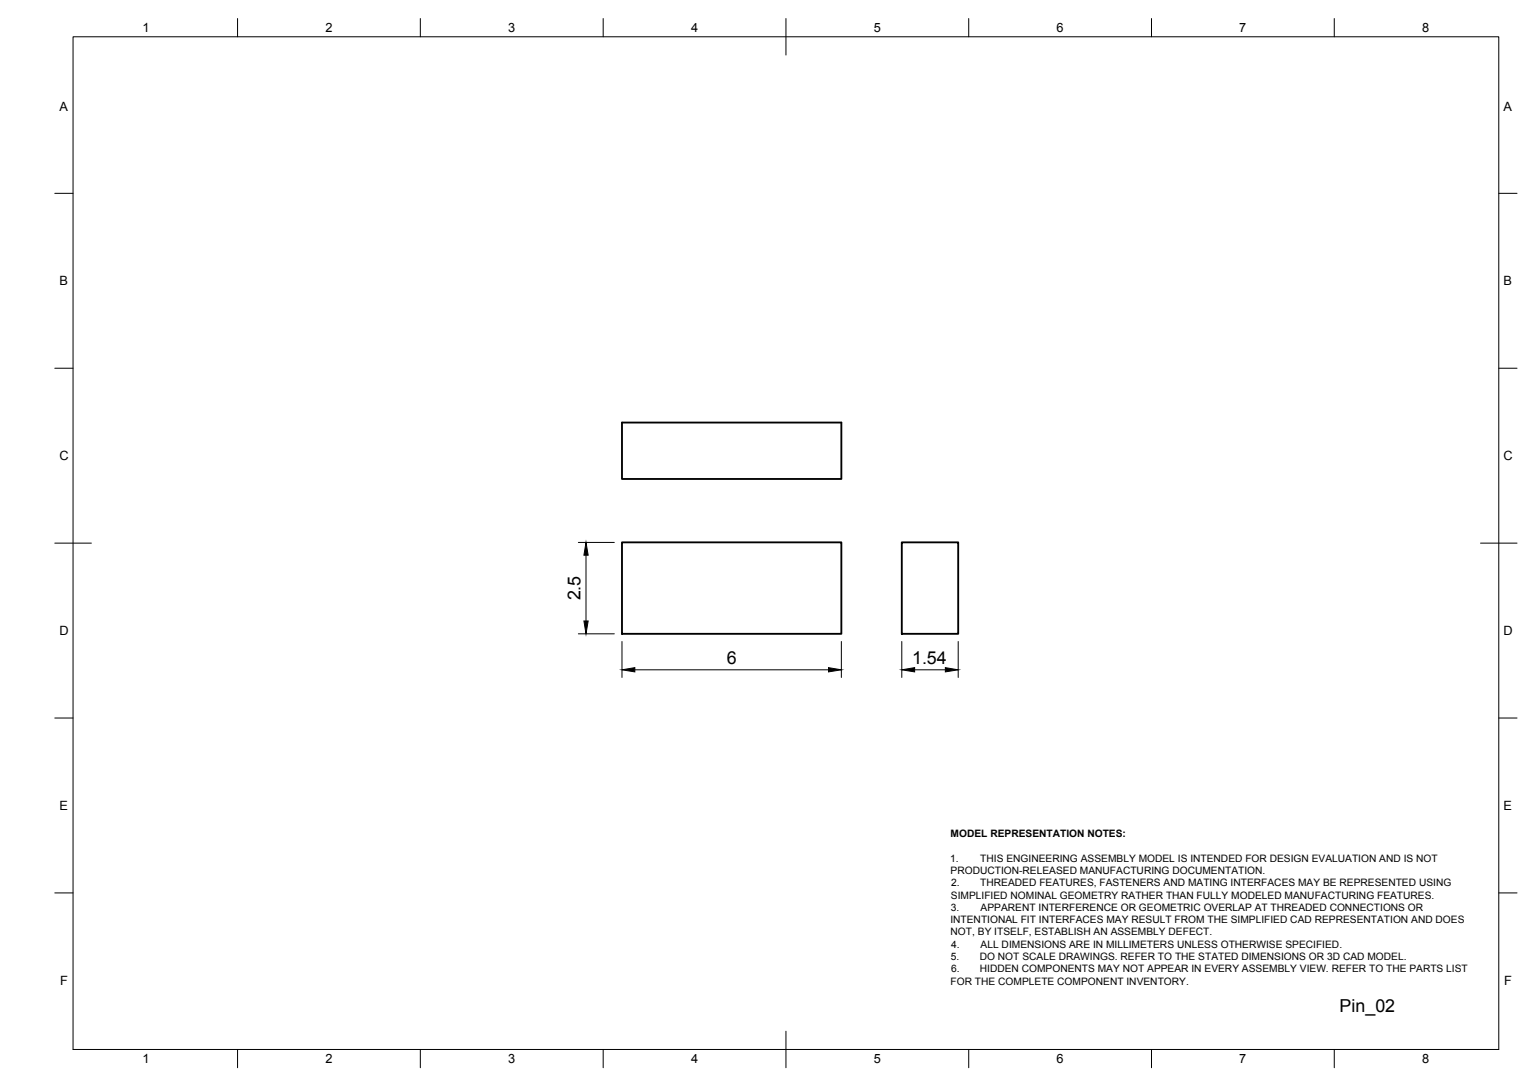
ISO-10303-21;
HEADER;
/* Generated by software containing ST-Developer
 * from STEP Tools, Inc. (www.steptools.com) 
 */

FILE_DESCRIPTION(
/* description */ (''),
/* implementation_level */ '2;1');

FILE_NAME(
/* name */ 'Pin_02.step',
/* time_stamp */ '2026-10-05T22:24:12-07:00',
/* author */ (''),
/* organization */ (''),
/* preprocessor_version */ 'ST-DEVELOPER v20.2',
/* originating_system */ 'Autodesk Translation Framework v15.15.0.0',
/* authorisation */ '');

FILE_SCHEMA (('AUTOMOTIVE_DESIGN { 1 0 10303 214 3 1 1 }'));
ENDSEC;

DATA;
#10=MECHANICAL_DESIGN_GEOMETRIC_PRESENTATION_REPRESENTATION('',(#57),#2116);
#43=SHAPE_REPRESENTATION_RELATIONSHIP('SRR','None',#2149,#50);
#50=ADVANCED_BREP_SHAPE_REPRESENTATION('',(#64),#2113);
#57=STYLED_ITEM('',(#2192),#64);
#64=MANIFOLD_SOLID_BREP('Body1',#1151);
#113=PLANE('',#1322);
#114=PLANE('',#1323);
#115=PLANE('',#1324);
#116=PLANE('',#1325);
#117=PLANE('',#1326);
#118=PLANE('',#1327);
#179=FACE_OUTER_BOUND('',#254,.T.);
#180=FACE_OUTER_BOUND('',#255,.T.);
#181=FACE_OUTER_BOUND('',#256,.T.);
#182=FACE_OUTER_BOUND('',#257,.T.);
#183=FACE_OUTER_BOUND('',#258,.T.);
#184=FACE_OUTER_BOUND('',#259,.T.);
#254=EDGE_LOOP('',(#991,#992,#993,#994));
#255=EDGE_LOOP('',(#995,#996,#997,#998));
#256=EDGE_LOOP('',(#999,#1000,#1001,#1002));
#257=EDGE_LOOP('',(#1003,#1004,#1005,#1006));
#258=EDGE_LOOP('',(#1007,#1008,#1009,#1010));
#259=EDGE_LOOP('',(#1011,#1012,#1013,#1014));
#346=LINE('',#2009,#451);
#347=LINE('',#2011,#452);
#348=LINE('',#2013,#453);
#349=LINE('',#2014,#454);
#350=LINE('',#2017,#455);
#351=LINE('',#2019,#456);
#352=LINE('',#2020,#457);
#353=LINE('',#2023,#458);
#354=LINE('',#2025,#459);
#355=LINE('',#2026,#460);
#356=LINE('',#2028,#461);
#357=LINE('',#2029,#462);
#451=VECTOR('',#1606,10.);
#452=VECTOR('',#1607,10.);
#453=VECTOR('',#1608,10.);
#454=VECTOR('',#1609,10.);
#455=VECTOR('',#1612,10.);
#456=VECTOR('',#1613,10.);
#457=VECTOR('',#1614,10.);
#458=VECTOR('',#1617,10.);
#459=VECTOR('',#1618,10.);
#460=VECTOR('',#1619,10.);
#461=VECTOR('',#1622,10.);
#462=VECTOR('',#1623,10.);
#599=VERTEX_POINT('',#2007);
#600=VERTEX_POINT('',#2008);
#601=VERTEX_POINT('',#2010);
#602=VERTEX_POINT('',#2012);
#603=VERTEX_POINT('',#2016);
#604=VERTEX_POINT('',#2018);
#605=VERTEX_POINT('',#2022);
#606=VERTEX_POINT('',#2024);
#734=EDGE_CURVE('',#599,#600,#346,.T.);
#735=EDGE_CURVE('',#600,#601,#347,.T.);
#736=EDGE_CURVE('',#601,#602,#348,.T.);
#737=EDGE_CURVE('',#599,#602,#349,.T.);
#738=EDGE_CURVE('',#600,#603,#350,.T.);
#739=EDGE_CURVE('',#603,#604,#351,.T.);
#740=EDGE_CURVE('',#604,#601,#352,.T.);
#741=EDGE_CURVE('',#605,#603,#353,.T.);
#742=EDGE_CURVE('',#605,#606,#354,.T.);
#743=EDGE_CURVE('',#606,#604,#355,.T.);
#744=EDGE_CURVE('',#599,#605,#356,.T.);
#745=EDGE_CURVE('',#602,#606,#357,.T.);
#991=ORIENTED_EDGE('',*,*,#734,.T.);
#992=ORIENTED_EDGE('',*,*,#735,.T.);
#993=ORIENTED_EDGE('',*,*,#736,.T.);
#994=ORIENTED_EDGE('',*,*,#737,.F.);
#995=ORIENTED_EDGE('',*,*,#738,.T.);
#996=ORIENTED_EDGE('',*,*,#739,.T.);
#997=ORIENTED_EDGE('',*,*,#740,.T.);
#998=ORIENTED_EDGE('',*,*,#735,.F.);
#999=ORIENTED_EDGE('',*,*,#741,.F.);
#1000=ORIENTED_EDGE('',*,*,#742,.T.);
#1001=ORIENTED_EDGE('',*,*,#743,.T.);
#1002=ORIENTED_EDGE('',*,*,#739,.F.);
#1003=ORIENTED_EDGE('',*,*,#744,.F.);
#1004=ORIENTED_EDGE('',*,*,#737,.T.);
#1005=ORIENTED_EDGE('',*,*,#745,.T.);
#1006=ORIENTED_EDGE('',*,*,#742,.F.);
#1007=ORIENTED_EDGE('',*,*,#745,.F.);
#1008=ORIENTED_EDGE('',*,*,#736,.F.);
#1009=ORIENTED_EDGE('',*,*,#740,.F.);
#1010=ORIENTED_EDGE('',*,*,#743,.F.);
#1011=ORIENTED_EDGE('',*,*,#744,.T.);
#1012=ORIENTED_EDGE('',*,*,#741,.T.);
#1013=ORIENTED_EDGE('',*,*,#738,.F.);
#1014=ORIENTED_EDGE('',*,*,#734,.F.);
#1128=ADVANCED_FACE('',(#179),#113,.F.);
#1129=ADVANCED_FACE('',(#180),#114,.F.);
#1130=ADVANCED_FACE('',(#181),#115,.F.);
#1131=ADVANCED_FACE('',(#182),#116,.F.);
#1132=ADVANCED_FACE('',(#183),#117,.F.);
#1133=ADVANCED_FACE('',(#184),#118,.T.);
#1151=CLOSED_SHELL('',(#1128,#1129,#1130,#1131,#1132,#1133));
#1321=AXIS2_PLACEMENT_3D('',#2005,#1602,#1603);
#1322=AXIS2_PLACEMENT_3D('',#2006,#1604,#1605);
#1323=AXIS2_PLACEMENT_3D('',#2015,#1610,#1611);
#1324=AXIS2_PLACEMENT_3D('',#2021,#1615,#1616);
#1325=AXIS2_PLACEMENT_3D('',#2027,#1620,#1621);
#1326=AXIS2_PLACEMENT_3D('',#2030,#1624,#1625);
#1327=AXIS2_PLACEMENT_3D('',#2031,#1626,#1627);
#1602=DIRECTION('axis',(0.,0.,1.));
#1603=DIRECTION('refdir',(1.,0.,0.));
#1604=DIRECTION('center_axis',(0.,0.,-1.));
#1605=DIRECTION('ref_axis',(-1.,0.,0.));
#1606=DIRECTION('',(1.,0.,0.));
#1607=DIRECTION('',(0.,1.,0.));
#1608=DIRECTION('',(-1.,0.,0.));
#1609=DIRECTION('',(0.,1.,0.));
#1610=DIRECTION('center_axis',(-1.,0.,0.));
#1611=DIRECTION('ref_axis',(0.,0.,1.));
#1612=DIRECTION('',(0.,0.,-1.));
#1613=DIRECTION('',(0.,1.,0.));
#1614=DIRECTION('',(0.,0.,1.));
#1615=DIRECTION('center_axis',(0.,0.,1.));
#1616=DIRECTION('ref_axis',(1.,0.,0.));
#1617=DIRECTION('',(1.,0.,0.));
#1618=DIRECTION('',(0.,1.,0.));
#1619=DIRECTION('',(1.,0.,0.));
#1620=DIRECTION('center_axis',(1.,0.,0.));
#1621=DIRECTION('ref_axis',(0.,0.,-1.));
#1622=DIRECTION('',(0.,0.,-1.));
#1623=DIRECTION('',(0.,0.,-1.));
#1624=DIRECTION('center_axis',(0.,-1.,0.));
#1625=DIRECTION('ref_axis',(0.,0.,-1.));
#1626=DIRECTION('center_axis',(0.,-1.,0.));
#1627=DIRECTION('ref_axis',(1.,0.,0.));
#2005=CARTESIAN_POINT('',(0.,0.,0.));
#2006=CARTESIAN_POINT('Origin',(3.25,10.,6.84122918275927));
#2007=CARTESIAN_POINT('',(0.75,10.,6.84122918275927));
#2008=CARTESIAN_POINT('',(3.25,10.,6.84122918275927));
#2009=CARTESIAN_POINT('',(0.75,10.,6.84122918275927));
#2010=CARTESIAN_POINT('',(3.25,16.,6.84122918275927));
#2011=CARTESIAN_POINT('',(3.25,10.,6.84122918275927));
#2012=CARTESIAN_POINT('',(0.75,16.,6.84122918275927));
#2013=CARTESIAN_POINT('',(0.75,16.,6.84122918275927));
#2014=CARTESIAN_POINT('',(0.75,10.,6.84122918275927));
#2015=CARTESIAN_POINT('Origin',(3.25,10.,5.29967103839267));
#2016=CARTESIAN_POINT('',(3.25,10.,5.29967103839267));
#2017=CARTESIAN_POINT('',(3.25,10.,8.32461990770089));
#2018=CARTESIAN_POINT('',(3.25,16.,5.29967103839267));
#2019=CARTESIAN_POINT('',(3.25,10.,5.29967103839267));
#2020=CARTESIAN_POINT('',(3.25,16.,8.32461990770089));
#2021=CARTESIAN_POINT('Origin',(0.75,10.,5.29967103839267));
#2022=CARTESIAN_POINT('',(0.75,10.,5.29967103839267));
#2023=CARTESIAN_POINT('',(0.75,10.,5.29967103839267));
#2024=CARTESIAN_POINT('',(0.75,16.,5.29967103839267));
#2025=CARTESIAN_POINT('',(0.75,10.,5.29967103839267));
#2026=CARTESIAN_POINT('',(0.75,16.,5.29967103839267));
#2027=CARTESIAN_POINT('Origin',(0.75,10.,6.84122918275927));
#2028=CARTESIAN_POINT('',(0.75,10.,5.79967103839267));
#2029=CARTESIAN_POINT('',(0.75,16.,5.79967103839267));
#2030=CARTESIAN_POINT('Origin',(2.,16.,6.07045011057597));
#2031=CARTESIAN_POINT('Origin',(2.,10.,6.07045011057597));
#2104=UNCERTAINTY_MEASURE_WITH_UNIT(LENGTH_MEASURE(0.01),#2117,
'DISTANCE_ACCURACY_VALUE',
'Maximum model space distance between geometric entities at asserted c
onnectivities');
#2107=UNCERTAINTY_MEASURE_WITH_UNIT(LENGTH_MEASURE(0.01),#2117,
'DISTANCE_ACCURACY_VALUE',
'Maximum model space distance between geometric entities at asserted c
onnectivities');
#2113=(
GEOMETRIC_REPRESENTATION_CONTEXT(3)
GLOBAL_UNCERTAINTY_ASSIGNED_CONTEXT((#2104))
GLOBAL_UNIT_ASSIGNED_CONTEXT((#2117,#2119,#2120))
REPRESENTATION_CONTEXT('','3D')
);
#2116=(
GEOMETRIC_REPRESENTATION_CONTEXT(3)
GLOBAL_UNCERTAINTY_ASSIGNED_CONTEXT((#2107))
GLOBAL_UNIT_ASSIGNED_CONTEXT((#2117,#2119,#2120))
REPRESENTATION_CONTEXT('','3D')
);
#2117=(
LENGTH_UNIT()
NAMED_UNIT(*)
SI_UNIT(.MILLI.,.METRE.)
);
#2119=(
NAMED_UNIT(*)
PLANE_ANGLE_UNIT()
SI_UNIT($,.RADIAN.)
);
#2120=(
NAMED_UNIT(*)
SI_UNIT($,.STERADIAN.)
SOLID_ANGLE_UNIT()
);
#2126=SHAPE_DEFINITION_REPRESENTATION(#2134,#2149);
#2134=PRODUCT_DEFINITION_SHAPE('',$,#2158);
#2149=SHAPE_REPRESENTATION('',(#1321),#2113);
#2152=PRODUCT_DEFINITION_CONTEXT('part definition',#2178,'design');
#2158=PRODUCT_DEFINITION('Pin_02','Pin_02',#2166,#2152);
#2166=PRODUCT_DEFINITION_FORMATION('',$,#2185);
#2178=APPLICATION_CONTEXT(
'Core Data for Automotive Mechanical Design Process');
#2179=PRODUCT_CONTEXT('part definition',#2178,'mechanical');
#2185=PRODUCT('Pin_02','Pin_02',$,(#2179));
#2192=PRESENTATION_STYLE_ASSIGNMENT((#2197));
#2197=SURFACE_STYLE_USAGE(.BOTH.,#2202);
#2202=SURFACE_SIDE_STYLE('',(#2207));
#2207=SURFACE_STYLE_FILL_AREA(#2212);
#2212=FILL_AREA_STYLE('Opaque(235,235,235)',(#2217));
#2217=FILL_AREA_STYLE_COLOUR('Opaque(235,235,235)',#2222);
#2222=COLOUR_RGB('Opaque(235,235,235)', 0.40784314, 0.44705882, 0.49803922);
ENDSEC;
END-ISO-10303-21;
